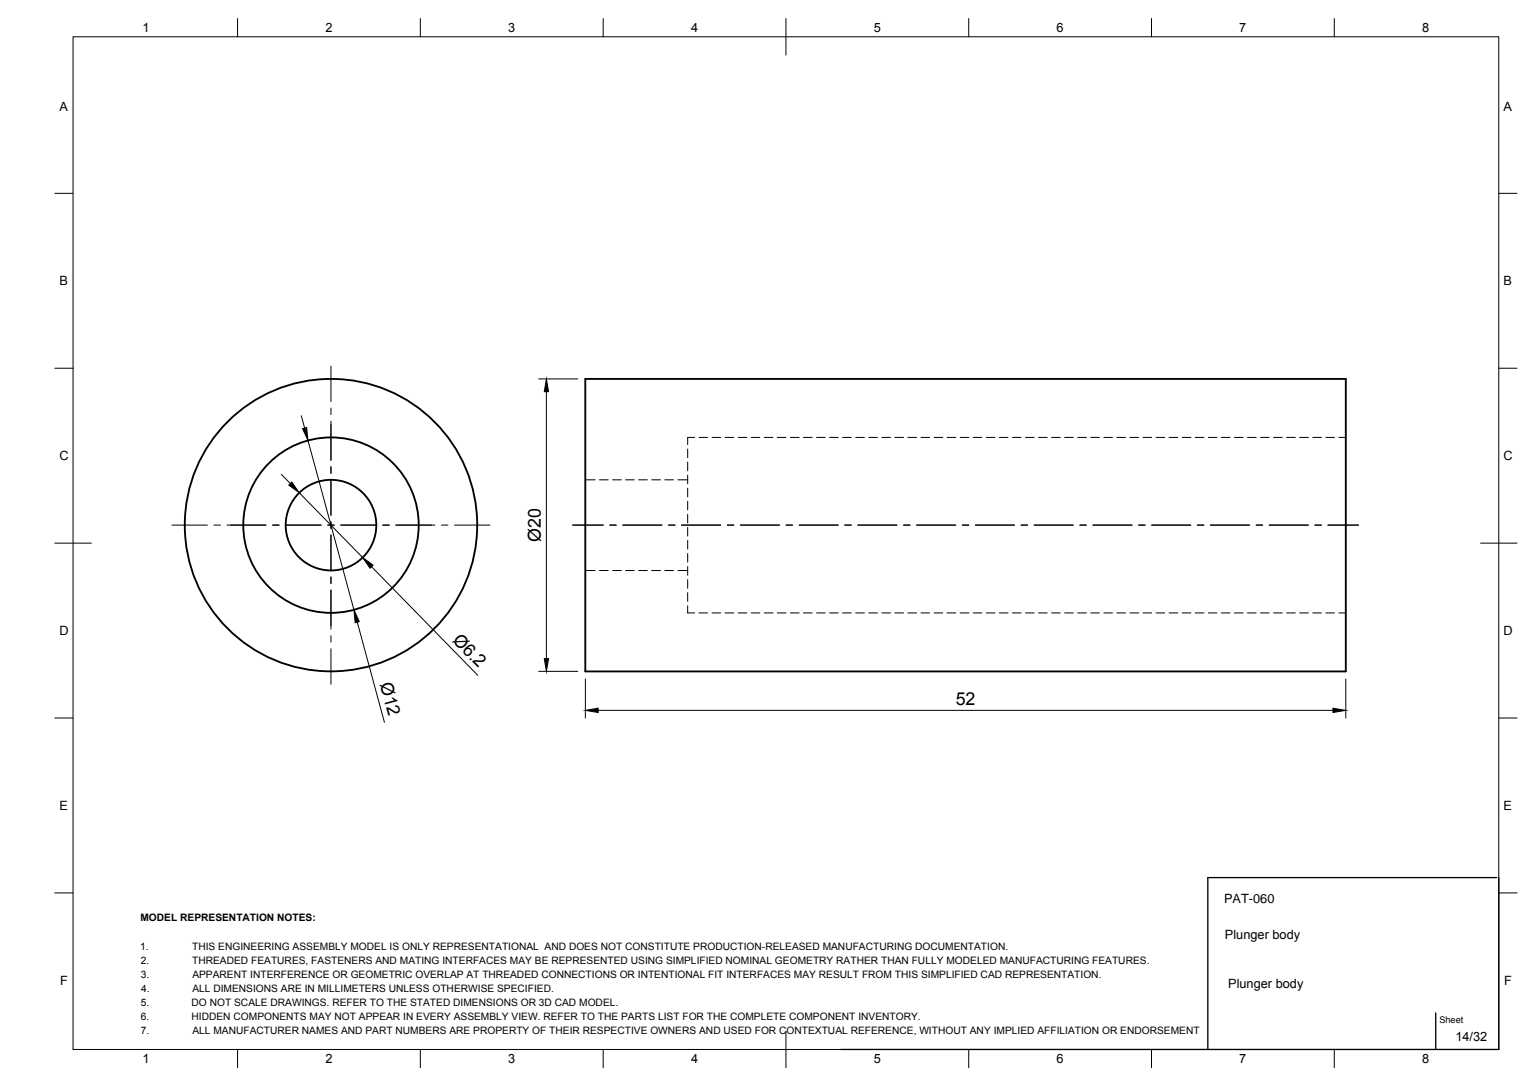
ISO-10303-21;
HEADER;
/* Generated by software containing ST-Developer
 * from STEP Tools, Inc. (www.steptools.com) 
 */

FILE_DESCRIPTION(
/* description */ ('Indexing fixture plate with plunger'),
/* implementation_level */ '2;1');

FILE_NAME(
/* name */ 'Plunger body.step',
/* time_stamp */ '2026-10-28T03:23:41-07:00',
/* author */ (''),
/* organization */ (''),
/* preprocessor_version */ 'ST-DEVELOPER v20.2',
/* originating_system */ 'Autodesk Translation Framework v15.17.0.0',
/* authorisation */ '');

FILE_SCHEMA (('AUTOMOTIVE_DESIGN { 1 0 10303 214 3 1 1 }'));
ENDSEC;

DATA;
#10=MECHANICAL_DESIGN_GEOMETRIC_PRESENTATION_REPRESENTATION('',(#326),#10020);
#272=SHAPE_REPRESENTATION_RELATIONSHIP('SRR','None',#10146,#299);
#299=ADVANCED_BREP_SHAPE_REPRESENTATION('',(#362),#9999);
#326=STYLED_ITEM('',(#10347),#362);
#362=MANIFOLD_SOLID_BREP('Body1',#4580);
#425=FACE_BOUND('',#1053,.T.);
#426=FACE_BOUND('',#1057,.T.);
#427=FACE_BOUND('',#1059,.T.);
#565=PLANE('',#5037);
#566=PLANE('',#5044);
#567=PLANE('',#5045);
#727=FACE_OUTER_BOUND('',#1051,.T.);
#728=FACE_OUTER_BOUND('',#1052,.T.);
#729=FACE_OUTER_BOUND('',#1054,.T.);
#730=FACE_OUTER_BOUND('',#1055,.T.);
#731=FACE_OUTER_BOUND('',#1056,.T.);
#732=FACE_OUTER_BOUND('',#1058,.T.);
#1051=EDGE_LOOP('',(#3275,#3276,#3277,#3278));
#1052=EDGE_LOOP('',(#3279));
#1053=EDGE_LOOP('',(#3280));
#1054=EDGE_LOOP('',(#3281,#3282,#3283,#3284));
#1055=EDGE_LOOP('',(#3285,#3286,#3287,#3288));
#1056=EDGE_LOOP('',(#3289));
#1057=EDGE_LOOP('',(#3290));
#1058=EDGE_LOOP('',(#3291));
#1059=EDGE_LOOP('',(#3292));
#1435=LINE('',#7436,#1655);
#1436=LINE('',#7443,#1656);
#1437=LINE('',#7449,#1657);
#1655=VECTOR('',#5874,0.31);
#1656=VECTOR('',#5883,0.6);
#1657=VECTOR('',#5890,0.999999999999999);
#1890=CIRCLE('',#5035,0.31);
#1891=CIRCLE('',#5036,0.31);
#1892=CIRCLE('',#5038,0.6);
#1893=CIRCLE('',#5040,0.6);
#1894=CIRCLE('',#5042,0.999999999999999);
#1895=CIRCLE('',#5043,0.999999999999999);
#2206=VERTEX_POINT('',#7433);
#2207=VERTEX_POINT('',#7435);
#2208=VERTEX_POINT('',#7439);
#2209=VERTEX_POINT('',#7442);
#2210=VERTEX_POINT('',#7446);
#2211=VERTEX_POINT('',#7448);
#2617=EDGE_CURVE('',#2206,#2206,#1890,.T.);
#2618=EDGE_CURVE('',#2206,#2207,#1435,.T.);
#2619=EDGE_CURVE('',#2207,#2207,#1891,.T.);
#2620=EDGE_CURVE('',#2208,#2208,#1892,.T.);
#2621=EDGE_CURVE('',#2208,#2209,#1436,.T.);
#2622=EDGE_CURVE('',#2209,#2209,#1893,.T.);
#2623=EDGE_CURVE('',#2210,#2210,#1894,.T.);
#2624=EDGE_CURVE('',#2210,#2211,#1437,.T.);
#2625=EDGE_CURVE('',#2211,#2211,#1895,.T.);
#3275=ORIENTED_EDGE('',*,*,#2617,.F.);
#3276=ORIENTED_EDGE('',*,*,#2618,.T.);
#3277=ORIENTED_EDGE('',*,*,#2619,.T.);
#3278=ORIENTED_EDGE('',*,*,#2618,.F.);
#3279=ORIENTED_EDGE('',*,*,#2620,.F.);
#3280=ORIENTED_EDGE('',*,*,#2619,.F.);
#3281=ORIENTED_EDGE('',*,*,#2620,.T.);
#3282=ORIENTED_EDGE('',*,*,#2621,.T.);
#3283=ORIENTED_EDGE('',*,*,#2622,.T.);
#3284=ORIENTED_EDGE('',*,*,#2621,.F.);
#3285=ORIENTED_EDGE('',*,*,#2623,.F.);
#3286=ORIENTED_EDGE('',*,*,#2624,.T.);
#3287=ORIENTED_EDGE('',*,*,#2625,.T.);
#3288=ORIENTED_EDGE('',*,*,#2624,.F.);
#3289=ORIENTED_EDGE('',*,*,#2623,.T.);
#3290=ORIENTED_EDGE('',*,*,#2617,.T.);
#3291=ORIENTED_EDGE('',*,*,#2625,.F.);
#3292=ORIENTED_EDGE('',*,*,#2622,.F.);
#4196=CYLINDRICAL_SURFACE('',#5034,0.31);
#4197=CYLINDRICAL_SURFACE('',#5039,0.6);
#4198=CYLINDRICAL_SURFACE('',#5041,0.999999999999999);
#4342=ADVANCED_FACE('',(#727),#4196,.F.);
#4343=ADVANCED_FACE('',(#728,#425),#565,.F.);
#4344=ADVANCED_FACE('',(#729),#4197,.F.);
#4345=ADVANCED_FACE('',(#730),#4198,.T.);
#4346=ADVANCED_FACE('',(#731,#426),#566,.T.);
#4347=ADVANCED_FACE('',(#732,#427),#567,.F.);
#4580=CLOSED_SHELL('',(#4342,#4343,#4344,#4345,#4346,#4347));
#5033=AXIS2_PLACEMENT_3D('',#7431,#5868,#5869);
#5034=AXIS2_PLACEMENT_3D('',#7432,#5870,#5871);
#5035=AXIS2_PLACEMENT_3D('',#7434,#5872,#5873);
#5036=AXIS2_PLACEMENT_3D('',#7437,#5875,#5876);
#5037=AXIS2_PLACEMENT_3D('',#7438,#5877,#5878);
#5038=AXIS2_PLACEMENT_3D('',#7440,#5879,#5880);
#5039=AXIS2_PLACEMENT_3D('',#7441,#5881,#5882);
#5040=AXIS2_PLACEMENT_3D('',#7444,#5884,#5885);
#5041=AXIS2_PLACEMENT_3D('',#7445,#5886,#5887);
#5042=AXIS2_PLACEMENT_3D('',#7447,#5888,#5889);
#5043=AXIS2_PLACEMENT_3D('',#7450,#5891,#5892);
#5044=AXIS2_PLACEMENT_3D('',#7451,#5893,#5894);
#5045=AXIS2_PLACEMENT_3D('',#7452,#5895,#5896);
#5868=DIRECTION('axis',(0.,0.,1.));
#5869=DIRECTION('refdir',(1.,0.,0.));
#5870=DIRECTION('center_axis',(0.,0.,1.));
#5871=DIRECTION('ref_axis',(1.,0.,0.));
#5872=DIRECTION('center_axis',(0.,0.,-1.));
#5873=DIRECTION('ref_axis',(1.,0.,0.));
#5874=DIRECTION('',(0.,0.,-1.));
#5875=DIRECTION('center_axis',(0.,0.,-1.));
#5876=DIRECTION('ref_axis',(1.,0.,0.));
#5877=DIRECTION('center_axis',(0.,0.,1.));
#5878=DIRECTION('ref_axis',(1.,0.,0.));
#5879=DIRECTION('center_axis',(0.,0.,1.));
#5880=DIRECTION('ref_axis',(1.,0.,0.));
#5881=DIRECTION('center_axis',(0.,0.,1.));
#5882=DIRECTION('ref_axis',(1.,0.,0.));
#5883=DIRECTION('',(0.,0.,-1.));
#5884=DIRECTION('center_axis',(0.,0.,-1.));
#5885=DIRECTION('ref_axis',(1.,0.,0.));
#5886=DIRECTION('center_axis',(0.,0.,1.));
#5887=DIRECTION('ref_axis',(1.,0.,0.));
#5888=DIRECTION('center_axis',(0.,0.,1.));
#5889=DIRECTION('ref_axis',(1.,0.,0.));
#5890=DIRECTION('',(0.,0.,-1.));
#5891=DIRECTION('center_axis',(0.,0.,1.));
#5892=DIRECTION('ref_axis',(1.,0.,0.));
#5893=DIRECTION('center_axis',(0.,0.,1.));
#5894=DIRECTION('ref_axis',(1.,0.,0.));
#5895=DIRECTION('center_axis',(0.,0.,1.));
#5896=DIRECTION('ref_axis',(1.,0.,0.));
#7431=CARTESIAN_POINT('',(0.,0.,0.));
#7432=CARTESIAN_POINT('Origin',(7.2,0.,5.));
#7433=CARTESIAN_POINT('',(6.89,-3.79640507735679E-17,5.7));
#7434=CARTESIAN_POINT('Origin',(7.2,0.,5.7));
#7435=CARTESIAN_POINT('',(6.89,-3.79640507735679E-17,5.));
#7436=CARTESIAN_POINT('',(6.89,-3.79640507735679E-17,5.));
#7437=CARTESIAN_POINT('Origin',(7.2,0.,5.));
#7438=CARTESIAN_POINT('Origin',(7.2,0.,5.));
#7439=CARTESIAN_POINT('',(6.6,-7.34788079488412E-17,5.));
#7440=CARTESIAN_POINT('Origin',(7.2,0.,5.));
#7441=CARTESIAN_POINT('Origin',(7.2,0.,0.5));
#7442=CARTESIAN_POINT('',(6.6,-7.34788079488412E-17,0.5));
#7443=CARTESIAN_POINT('',(6.6,-7.34788079488412E-17,0.5));
#7444=CARTESIAN_POINT('Origin',(7.2,0.,0.5));
#7445=CARTESIAN_POINT('Origin',(7.2,0.,0.5));
#7446=CARTESIAN_POINT('',(6.2,-1.22464679914735E-16,5.7));
#7447=CARTESIAN_POINT('Origin',(7.2,0.,5.7));
#7448=CARTESIAN_POINT('',(6.2,-1.22464679914735E-16,0.5));
#7449=CARTESIAN_POINT('',(6.2,-1.22464679914735E-16,0.5));
#7450=CARTESIAN_POINT('Origin',(7.2,0.,0.5));
#7451=CARTESIAN_POINT('Origin',(7.2,0.,5.7));
#7452=CARTESIAN_POINT('Origin',(7.2,0.,0.5));
#9966=UNCERTAINTY_MEASURE_WITH_UNIT(LENGTH_MEASURE(0.001),#10021,
'DISTANCE_ACCURACY_VALUE',
'Maximum model space distance between geometric entities at asserted c
onnectivities');
#9987=UNCERTAINTY_MEASURE_WITH_UNIT(LENGTH_MEASURE(0.001),#10021,
'DISTANCE_ACCURACY_VALUE',
'Maximum model space distance between geometric entities at asserted c
onnectivities');
#9999=(
GEOMETRIC_REPRESENTATION_CONTEXT(3)
GLOBAL_UNCERTAINTY_ASSIGNED_CONTEXT((#9966))
GLOBAL_UNIT_ASSIGNED_CONTEXT((#10021,#10023,#10024))
REPRESENTATION_CONTEXT('','3D')
);
#10020=(
GEOMETRIC_REPRESENTATION_CONTEXT(3)
GLOBAL_UNCERTAINTY_ASSIGNED_CONTEXT((#9987))
GLOBAL_UNIT_ASSIGNED_CONTEXT((#10021,#10023,#10024))
REPRESENTATION_CONTEXT('','3D')
);
#10021=(
LENGTH_UNIT()
NAMED_UNIT(*)
SI_UNIT(.CENTI.,.METRE.)
);
#10023=(
NAMED_UNIT(*)
PLANE_ANGLE_UNIT()
SI_UNIT($,.RADIAN.)
);
#10024=(
NAMED_UNIT(*)
SI_UNIT($,.STERADIAN.)
SOLID_ANGLE_UNIT()
);
#10036=SHAPE_DEFINITION_REPRESENTATION(#10068,#10146);
#10068=PRODUCT_DEFINITION_SHAPE('',$,#10179);
#10146=SHAPE_REPRESENTATION('',(#5033),#9999);
#10167=PRODUCT_DEFINITION_CONTEXT('part definition',#10265,'design');
#10179=PRODUCT_DEFINITION('Plunger body','Plunger body',#10211,#10167);
#10211=PRODUCT_DEFINITION_FORMATION('',$,#10278);
#10265=APPLICATION_CONTEXT(
'Core Data for Automotive Mechanical Design Process');
#10266=PRODUCT_CONTEXT('part definition',#10265,'mechanical');
#10278=PRODUCT('Plunger body','Plunger body','Plunger body',(#10266));
#10341=COLOUR_RGB('Dark Blue',0.08,0.2,0.34);
#10342=FILL_AREA_STYLE_COLOUR('',#10341);
#10343=FILL_AREA_STYLE('',(#10342));
#10344=SURFACE_STYLE_FILL_AREA(#10343);
#10345=SURFACE_SIDE_STYLE('',(#10344));
#10346=SURFACE_STYLE_USAGE(.BOTH.,#10345);
#10347=PRESENTATION_STYLE_ASSIGNMENT((#10346));
ENDSEC;
END-ISO-10303-21;
